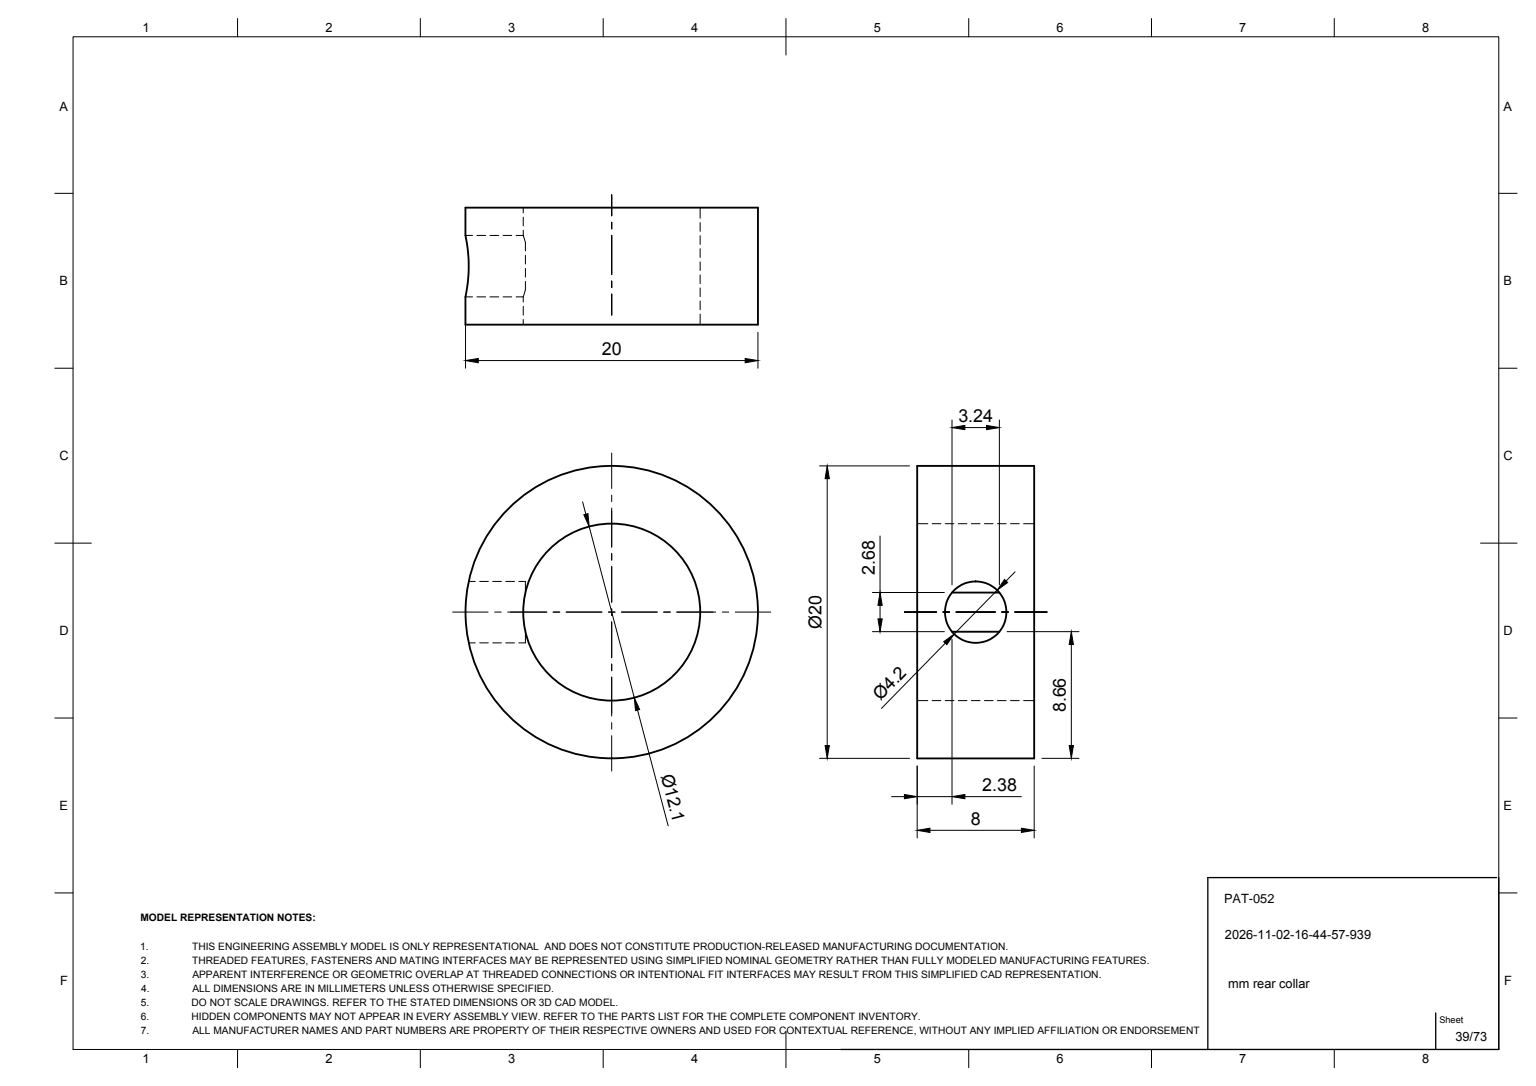
ISO-10303-21;
HEADER;
/* Generated by software containing ST-Developer
 * from STEP Tools, Inc. (www.steptools.com) 
 */

FILE_DESCRIPTION(
/* description */ ('Hand-crank gear train demonstrator'),
/* implementation_level */ '2;1');

FILE_NAME(
/* name */ 'mm rear collar.step',
/* time_stamp */ '2026-10-28T03:22:13-07:00',
/* author */ (''),
/* organization */ (''),
/* preprocessor_version */ 'ST-DEVELOPER v20.2',
/* originating_system */ 'Autodesk Translation Framework v15.17.0.0',
/* authorisation */ '');

FILE_SCHEMA (('AUTOMOTIVE_DESIGN { 1 0 10303 214 3 1 1 }'));
ENDSEC;

DATA;
#10=MECHANICAL_DESIGN_GEOMETRIC_PRESENTATION_REPRESENTATION('',(#1235),#62758);
#891=B_SPLINE_CURVE_WITH_KNOTS('',3,(#26102,#26103,#26104,#26105,#26106,
#26107,#26108,#26109,#26110,#26111),.UNSPECIFIED.,.F.,.F.,(4,2,2,2,4),(0.818088904349178,
0.878131747417164,0.957937926194035,1.03774410497091,1.09778694803889),
 .UNSPECIFIED.);
#892=B_SPLINE_CURVE_WITH_KNOTS('',3,(#26117,#26118,#26119,#26120,#26121,
#26122,#26123,#26124,#26125,#26126,#26127,#26128,#26129,#26130,#26131,#26132,
#26133,#26134),.UNSPECIFIED.,.F.,.F.,(4,2,2,2,2,2,2,2,4),(0.,0.0793616477694785,
0.158723295538957,0.238079516586307,0.317435737633656,0.396791958681006,
0.476148179728355,0.555509827497834,0.634871475267312),.UNSPECIFIED.);
#893=B_SPLINE_CURVE_WITH_KNOTS('',3,(#26135,#26136,#26137,#26138,#26139,
#26140,#26141,#26142,#26143,#26144,#26145,#26146,#26147,#26148,#26149,#26150,
#26151,#26152),.UNSPECIFIED.,.F.,.F.,(4,2,2,2,2,2,2,2,4),(0.634871475267312,
0.714233123036791,0.793594770806269,0.872950991853619,0.952307212900969,
1.03166343394832,1.11101965499567,1.19038130276515,1.26974295053462),
 .UNSPECIFIED.);
#894=B_SPLINE_CURVE_WITH_KNOTS('',3,(#26155,#26156,#26157,#26158,#26159,
#26160,#26161,#26162,#26163,#26164),.UNSPECIFIED.,.F.,.F.,(4,2,2,2,4),(0.179463620219821,
0.239506463287807,0.319312642064678,0.399118820841549,0.459161663909536),
 .UNSPECIFIED.);
#1092=SHAPE_REPRESENTATION_RELATIONSHIP('SRR','None',#63067,#1156);
#1156=ADVANCED_BREP_SHAPE_REPRESENTATION('',(#1311),#62721);
#1235=STYLED_ITEM('',(#63448),#1311);
#1311=MANIFOLD_SOLID_BREP('Body1',#16418);
#1551=FACE_BOUND('',#3723,.T.);
#1552=FACE_BOUND('',#3725,.T.);
#1553=FACE_BOUND('',#3727,.T.);
#1554=FACE_BOUND('',#3729,.T.);
#1902=PLANE('',#18024);
#1903=PLANE('',#18029);
#1904=PLANE('',#18036);
#1905=PLANE('',#18037);
#2574=FACE_OUTER_BOUND('',#3719,.T.);
#2575=FACE_OUTER_BOUND('',#3720,.T.);
#2576=FACE_OUTER_BOUND('',#3721,.T.);
#2577=FACE_OUTER_BOUND('',#3722,.T.);
#2578=FACE_OUTER_BOUND('',#3724,.T.);
#2579=FACE_OUTER_BOUND('',#3726,.T.);
#2580=FACE_OUTER_BOUND('',#3728,.T.);
#3719=EDGE_LOOP('',(#12805,#12806));
#3720=EDGE_LOOP('',(#12807,#12808,#12809,#12810,#12811,#12812,#12813,#12814,
#12815));
#3721=EDGE_LOOP('',(#12816,#12817,#12818));
#3722=EDGE_LOOP('',(#12819,#12820,#12821,#12822));
#3723=EDGE_LOOP('',(#12823,#12824,#12825,#12826));
#3724=EDGE_LOOP('',(#12827,#12828,#12829,#12830));
#3725=EDGE_LOOP('',(#12831,#12832));
#3726=EDGE_LOOP('',(#12833));
#3727=EDGE_LOOP('',(#12834));
#3728=EDGE_LOOP('',(#12835));
#3729=EDGE_LOOP('',(#12836));
#4871=LINE('',#26098,#6003);
#4872=LINE('',#26115,#6004);
#4873=LINE('',#26166,#6005);
#4874=LINE('',#26171,#6006);
#4875=LINE('',#26177,#6007);
#6003=VECTOR('',#21150,1.);
#6004=VECTOR('',#21157,0.21);
#6005=VECTOR('',#21162,1.);
#6006=VECTOR('',#21167,0.605);
#6007=VECTOR('',#21174,1.);
#6918=CIRCLE('',#18025,0.21);
#6919=CIRCLE('',#18027,0.21);
#6920=CIRCLE('',#18028,0.21);
#6921=CIRCLE('',#18031,0.605);
#6922=CIRCLE('',#18032,0.605);
#6923=CIRCLE('',#18034,1.);
#6924=CIRCLE('',#18035,1.);
#7883=VERTEX_POINT('',#26096);
#7884=VERTEX_POINT('',#26097);
#7885=VERTEX_POINT('',#26101);
#7886=VERTEX_POINT('',#26112);
#7887=VERTEX_POINT('',#26114);
#7888=VERTEX_POINT('',#26116);
#7889=VERTEX_POINT('',#26153);
#7890=VERTEX_POINT('',#26168);
#7891=VERTEX_POINT('',#26170);
#7892=VERTEX_POINT('',#26174);
#7893=VERTEX_POINT('',#26176);
#9654=EDGE_CURVE('',#7883,#7884,#4871,.T.);
#9655=EDGE_CURVE('',#7883,#7884,#6918,.T.);
#9656=EDGE_CURVE('',#7885,#7883,#891,.T.);
#9657=EDGE_CURVE('',#7886,#7885,#6919,.T.);
#9658=EDGE_CURVE('',#7886,#7887,#4872,.T.);
#9659=EDGE_CURVE('',#7888,#7887,#892,.T.);
#9660=EDGE_CURVE('',#7887,#7888,#893,.T.);
#9661=EDGE_CURVE('',#7889,#7886,#6920,.T.);
#9662=EDGE_CURVE('',#7884,#7889,#894,.T.);
#9663=EDGE_CURVE('',#7889,#7885,#4873,.T.);
#9664=EDGE_CURVE('',#7890,#7890,#6921,.T.);
#9665=EDGE_CURVE('',#7890,#7891,#4874,.T.);
#9666=EDGE_CURVE('',#7891,#7891,#6922,.T.);
#9667=EDGE_CURVE('',#7892,#7892,#6923,.T.);
#9668=EDGE_CURVE('',#7892,#7893,#4875,.T.);
#9669=EDGE_CURVE('',#7893,#7893,#6924,.T.);
#12805=ORIENTED_EDGE('',*,*,#9654,.F.);
#12806=ORIENTED_EDGE('',*,*,#9655,.T.);
#12807=ORIENTED_EDGE('',*,*,#9656,.F.);
#12808=ORIENTED_EDGE('',*,*,#9657,.F.);
#12809=ORIENTED_EDGE('',*,*,#9658,.T.);
#12810=ORIENTED_EDGE('',*,*,#9659,.F.);
#12811=ORIENTED_EDGE('',*,*,#9660,.F.);
#12812=ORIENTED_EDGE('',*,*,#9658,.F.);
#12813=ORIENTED_EDGE('',*,*,#9661,.F.);
#12814=ORIENTED_EDGE('',*,*,#9662,.F.);
#12815=ORIENTED_EDGE('',*,*,#9655,.F.);
#12816=ORIENTED_EDGE('',*,*,#9663,.F.);
#12817=ORIENTED_EDGE('',*,*,#9661,.T.);
#12818=ORIENTED_EDGE('',*,*,#9657,.T.);
#12819=ORIENTED_EDGE('',*,*,#9664,.F.);
#12820=ORIENTED_EDGE('',*,*,#9665,.T.);
#12821=ORIENTED_EDGE('',*,*,#9666,.T.);
#12822=ORIENTED_EDGE('',*,*,#9665,.F.);
#12823=ORIENTED_EDGE('',*,*,#9662,.T.);
#12824=ORIENTED_EDGE('',*,*,#9663,.T.);
#12825=ORIENTED_EDGE('',*,*,#9656,.T.);
#12826=ORIENTED_EDGE('',*,*,#9654,.T.);
#12827=ORIENTED_EDGE('',*,*,#9667,.F.);
#12828=ORIENTED_EDGE('',*,*,#9668,.T.);
#12829=ORIENTED_EDGE('',*,*,#9669,.T.);
#12830=ORIENTED_EDGE('',*,*,#9668,.F.);
#12831=ORIENTED_EDGE('',*,*,#9659,.T.);
#12832=ORIENTED_EDGE('',*,*,#9660,.T.);
#12833=ORIENTED_EDGE('',*,*,#9667,.T.);
#12834=ORIENTED_EDGE('',*,*,#9664,.T.);
#12835=ORIENTED_EDGE('',*,*,#9669,.F.);
#12836=ORIENTED_EDGE('',*,*,#9666,.F.);
#15298=CYLINDRICAL_SURFACE('',#18026,0.21);
#15299=CYLINDRICAL_SURFACE('',#18030,0.605);
#15300=CYLINDRICAL_SURFACE('',#18033,1.);
#15884=ADVANCED_FACE('',(#2574),#1902,.T.);
#15885=ADVANCED_FACE('',(#2575),#15298,.F.);
#15886=ADVANCED_FACE('',(#2576),#1903,.T.);
#15887=ADVANCED_FACE('',(#2577,#1551),#15299,.F.);
#15888=ADVANCED_FACE('',(#2578,#1552),#15300,.T.);
#15889=ADVANCED_FACE('',(#2579,#1553),#1904,.T.);
#15890=ADVANCED_FACE('',(#2580,#1554),#1905,.F.);
#16418=CLOSED_SHELL('',(#15884,#15885,#15886,#15887,#15888,#15889,#15890));
#18023=AXIS2_PLACEMENT_3D('',#26094,#21146,#21147);
#18024=AXIS2_PLACEMENT_3D('',#26095,#21148,#21149);
#18025=AXIS2_PLACEMENT_3D('',#26099,#21151,#21152);
#18026=AXIS2_PLACEMENT_3D('',#26100,#21153,#21154);
#18027=AXIS2_PLACEMENT_3D('',#26113,#21155,#21156);
#18028=AXIS2_PLACEMENT_3D('',#26154,#21158,#21159);
#18029=AXIS2_PLACEMENT_3D('',#26165,#21160,#21161);
#18030=AXIS2_PLACEMENT_3D('',#26167,#21163,#21164);
#18031=AXIS2_PLACEMENT_3D('',#26169,#21165,#21166);
#18032=AXIS2_PLACEMENT_3D('',#26172,#21168,#21169);
#18033=AXIS2_PLACEMENT_3D('',#26173,#21170,#21171);
#18034=AXIS2_PLACEMENT_3D('',#26175,#21172,#21173);
#18035=AXIS2_PLACEMENT_3D('',#26178,#21175,#21176);
#18036=AXIS2_PLACEMENT_3D('',#26179,#21177,#21178);
#18037=AXIS2_PLACEMENT_3D('',#26180,#21179,#21180);
#21146=DIRECTION('axis',(0.,0.,1.));
#21147=DIRECTION('refdir',(1.,0.,0.));
#21148=DIRECTION('center_axis',(0.,0.,1.));
#21149=DIRECTION('ref_axis',(1.,0.,0.));
#21150=DIRECTION('',(0.,1.,0.));
#21151=DIRECTION('center_axis',(0.,0.,1.));
#21152=DIRECTION('ref_axis',(1.,0.,0.));
#21153=DIRECTION('center_axis',(0.,0.,1.));
#21154=DIRECTION('ref_axis',(1.,0.,0.));
#21155=DIRECTION('center_axis',(0.,0.,1.));
#21156=DIRECTION('ref_axis',(1.,0.,0.));
#21157=DIRECTION('',(0.,0.,1.));
#21158=DIRECTION('center_axis',(0.,0.,1.));
#21159=DIRECTION('ref_axis',(1.,0.,0.));
#21160=DIRECTION('center_axis',(0.,0.,1.));
#21161=DIRECTION('ref_axis',(1.,0.,0.));
#21162=DIRECTION('',(0.,-1.,0.));
#21163=DIRECTION('center_axis',(0.,1.,0.));
#21164=DIRECTION('ref_axis',(1.,0.,0.));
#21165=DIRECTION('center_axis',(0.,-1.,0.));
#21166=DIRECTION('ref_axis',(1.,0.,0.));
#21167=DIRECTION('',(0.,-1.,0.));
#21168=DIRECTION('center_axis',(0.,-1.,0.));
#21169=DIRECTION('ref_axis',(1.,0.,0.));
#21170=DIRECTION('center_axis',(0.,1.,0.));
#21171=DIRECTION('ref_axis',(1.,0.,0.));
#21172=DIRECTION('center_axis',(0.,1.,0.));
#21173=DIRECTION('ref_axis',(1.,0.,0.));
#21174=DIRECTION('',(0.,-1.,0.));
#21175=DIRECTION('center_axis',(0.,1.,0.));
#21176=DIRECTION('ref_axis',(1.,0.,0.));
#21177=DIRECTION('center_axis',(0.,1.,0.));
#21178=DIRECTION('ref_axis',(1.,0.,0.));
#21179=DIRECTION('center_axis',(0.,1.,0.));
#21180=DIRECTION('ref_axis',(1.,0.,0.));
#26094=CARTESIAN_POINT('',(0.,0.,0.));
#26095=CARTESIAN_POINT('Origin',(0.,-3.2,9.59));
#26096=CARTESIAN_POINT('',(0.133884278389952,-3.36178689687364,9.59));
#26097=CARTESIAN_POINT('',(0.133884278389952,-3.03821310312636,9.59));
#26098=CARTESIAN_POINT('',(0.133884278389952,-3.6,9.59));
#26099=CARTESIAN_POINT('Origin',(0.,-3.2,9.59));
#26100=CARTESIAN_POINT('Origin',(0.,-3.2,9.59));
#26101=CARTESIAN_POINT('',(-0.133884278389952,-3.36178689687364,9.59));
#26102=CARTESIAN_POINT('Ctrl Pts',(-0.133884278389951,-3.36178689687364,
9.59));
#26103=CARTESIAN_POINT('Ctrl Pts',(-0.118254395260798,-3.37472116821763,
9.59354677224418));
#26104=CARTESIAN_POINT('Ctrl Pts',(-0.100109787682297,-3.38579931658744,
9.59698224789957));
#26105=CARTESIAN_POINT('Ctrl Pts',(-0.054829872132519,-3.40463856105443,
9.6030741628997));
#26106=CARTESIAN_POINT('Ctrl Pts',(-0.0266020595922904,-3.41,9.605));
#26107=CARTESIAN_POINT('Ctrl Pts',(0.0266020595922903,-3.41,9.605));
#26108=CARTESIAN_POINT('Ctrl Pts',(0.0548298721325192,-3.40463856105443,
9.6030741628997));
#26109=CARTESIAN_POINT('Ctrl Pts',(0.100109787682297,-3.38579931658744,
9.59698224789957));
#26110=CARTESIAN_POINT('Ctrl Pts',(0.118254395260799,-3.37472116821763,
9.59354677224418));
#26111=CARTESIAN_POINT('Ctrl Pts',(0.133884278389952,-3.36178689687364,
9.59));
#26112=CARTESIAN_POINT('',(-0.21,-3.2,9.59));
#26113=CARTESIAN_POINT('Origin',(0.,-3.2,9.59));
#26114=CARTESIAN_POINT('',(-0.21,-3.2,9.97770138590472));
#26115=CARTESIAN_POINT('',(-0.21,-3.2,9.59));
#26116=CARTESIAN_POINT('',(0.21,-3.2,9.97770138590472));
#26117=CARTESIAN_POINT('Ctrl Pts',(0.21,-3.2,9.97770138590472));
#26118=CARTESIAN_POINT('Ctrl Pts',(0.21,-3.22645388258983,9.97770138590472));
#26119=CARTESIAN_POINT('Ctrl Pts',(0.204697017125528,-3.25461525830869,
9.97888646613217));
#26120=CARTESIAN_POINT('Ctrl Pts',(0.183241751515529,-3.30633042130174,
9.98312869991147));
#26121=CARTESIAN_POINT('Ctrl Pts',(0.167093586802906,-3.32989126129544,
9.98612044796649));
#26122=CARTESIAN_POINT('Ctrl Pts',(0.129892533236543,-3.36709231486181,
9.99170645156379));
#26123=CARTESIAN_POINT('Ctrl Pts',(0.106331154992714,-3.38324147510569,
9.99466914446598));
#26124=CARTESIAN_POINT('Ctrl Pts',(0.0546141143983532,-3.40469746372443,
9.99884449237241));
#26125=CARTESIAN_POINT('Ctrl Pts',(0.0264520736824499,-3.41,10.));
#26126=CARTESIAN_POINT('Ctrl Pts',(-0.0264520736824498,-3.41,10.));
#26127=CARTESIAN_POINT('Ctrl Pts',(-0.0546141143983531,-3.40469746372443,
9.99884449237241));
#26128=CARTESIAN_POINT('Ctrl Pts',(-0.106331154992714,-3.38324147510569,
9.99466914446598));
#26129=CARTESIAN_POINT('Ctrl Pts',(-0.129892533236543,-3.36709231486181,
9.99170645156379));
#26130=CARTESIAN_POINT('Ctrl Pts',(-0.167093586802906,-3.32989126129544,
9.98612044796649));
#26131=CARTESIAN_POINT('Ctrl Pts',(-0.183241751515529,-3.30633042130174,
9.98312869991147));
#26132=CARTESIAN_POINT('Ctrl Pts',(-0.204697017125528,-3.25461525830869,
9.97888646613217));
#26133=CARTESIAN_POINT('Ctrl Pts',(-0.21,-3.22645388258983,9.97770138590472));
#26134=CARTESIAN_POINT('Ctrl Pts',(-0.21,-3.2,9.97770138590472));
#26135=CARTESIAN_POINT('Ctrl Pts',(-0.21,-3.2,9.97770138590472));
#26136=CARTESIAN_POINT('Ctrl Pts',(-0.21,-3.17354611741017,9.97770138590472));
#26137=CARTESIAN_POINT('Ctrl Pts',(-0.204697017125528,-3.14538474169131,
9.97888646613217));
#26138=CARTESIAN_POINT('Ctrl Pts',(-0.183241751515529,-3.09366957869826,
9.98312869991147));
#26139=CARTESIAN_POINT('Ctrl Pts',(-0.167093586802906,-3.07010873870456,
9.98612044796649));
#26140=CARTESIAN_POINT('Ctrl Pts',(-0.129892533236543,-3.03290768513819,
9.99170645156379));
#26141=CARTESIAN_POINT('Ctrl Pts',(-0.106331154992714,-3.01675852489431,
9.99466914446598));
#26142=CARTESIAN_POINT('Ctrl Pts',(-0.0546141143983532,-2.99530253627557,
9.99884449237241));
#26143=CARTESIAN_POINT('Ctrl Pts',(-0.0264520736824499,-2.99,10.));
#26144=CARTESIAN_POINT('Ctrl Pts',(0.0264520736824498,-2.99,10.));
#26145=CARTESIAN_POINT('Ctrl Pts',(0.0546141143983531,-2.99530253627557,
9.99884449237241));
#26146=CARTESIAN_POINT('Ctrl Pts',(0.106331154992714,-3.01675852489431,
9.99466914446598));
#26147=CARTESIAN_POINT('Ctrl Pts',(0.129892533236543,-3.03290768513819,
9.99170645156379));
#26148=CARTESIAN_POINT('Ctrl Pts',(0.167093586802906,-3.07010873870456,
9.98612044796649));
#26149=CARTESIAN_POINT('Ctrl Pts',(0.183241751515529,-3.09366957869826,
9.98312869991147));
#26150=CARTESIAN_POINT('Ctrl Pts',(0.204697017125528,-3.14538474169131,
9.97888646613217));
#26151=CARTESIAN_POINT('Ctrl Pts',(0.21,-3.17354611741017,9.97770138590472));
#26152=CARTESIAN_POINT('Ctrl Pts',(0.21,-3.2,9.97770138590472));
#26153=CARTESIAN_POINT('',(-0.133884278389952,-3.03821310312636,9.59));
#26154=CARTESIAN_POINT('Origin',(0.,-3.2,9.59));
#26155=CARTESIAN_POINT('Ctrl Pts',(0.133884278389952,-3.03821310312636,
9.59));
#26156=CARTESIAN_POINT('Ctrl Pts',(0.118254395260799,-3.02527883178237,
9.59354677224418));
#26157=CARTESIAN_POINT('Ctrl Pts',(0.100109787682297,-3.01420068341256,
9.59698224789957));
#26158=CARTESIAN_POINT('Ctrl Pts',(0.054829872132519,-2.99536143894557,
9.6030741628997));
#26159=CARTESIAN_POINT('Ctrl Pts',(0.0266020595922904,-2.99,9.605));
#26160=CARTESIAN_POINT('Ctrl Pts',(-0.0266020595922903,-2.99,9.605));
#26161=CARTESIAN_POINT('Ctrl Pts',(-0.054829872132519,-2.99536143894557,
9.6030741628997));
#26162=CARTESIAN_POINT('Ctrl Pts',(-0.100109787682297,-3.01420068341256,
9.59698224789957));
#26163=CARTESIAN_POINT('Ctrl Pts',(-0.118254395260798,-3.02527883178237,
9.59354677224418));
#26164=CARTESIAN_POINT('Ctrl Pts',(-0.133884278389952,-3.03821310312636,
9.59));
#26165=CARTESIAN_POINT('Origin',(0.,-3.2,9.59));
#26166=CARTESIAN_POINT('',(-0.133884278389952,-3.6,9.59));
#26167=CARTESIAN_POINT('Origin',(0.,-3.6,9.));
#26168=CARTESIAN_POINT('',(-0.605,-2.8,9.));
#26169=CARTESIAN_POINT('Origin',(0.,-2.8,9.));
#26170=CARTESIAN_POINT('',(-0.605,-3.6,9.));
#26171=CARTESIAN_POINT('',(-0.605,-3.6,9.));
#26172=CARTESIAN_POINT('Origin',(0.,-3.6,9.));
#26173=CARTESIAN_POINT('Origin',(0.,-3.6,9.));
#26174=CARTESIAN_POINT('',(-1.,-2.8,9.));
#26175=CARTESIAN_POINT('Origin',(0.,-2.8,9.));
#26176=CARTESIAN_POINT('',(-1.,-3.6,9.));
#26177=CARTESIAN_POINT('',(-1.,-3.6,9.));
#26178=CARTESIAN_POINT('Origin',(0.,-3.6,9.));
#26179=CARTESIAN_POINT('Origin',(0.,-2.8,9.));
#26180=CARTESIAN_POINT('Origin',(0.,-3.6,9.));
#62647=UNCERTAINTY_MEASURE_WITH_UNIT(LENGTH_MEASURE(0.001),#62759,
'DISTANCE_ACCURACY_VALUE',
'Maximum model space distance between geometric entities at asserted c
onnectivities');
#62684=UNCERTAINTY_MEASURE_WITH_UNIT(LENGTH_MEASURE(0.001),#62759,
'DISTANCE_ACCURACY_VALUE',
'Maximum model space distance between geometric entities at asserted c
onnectivities');
#62721=(
GEOMETRIC_REPRESENTATION_CONTEXT(3)
GLOBAL_UNCERTAINTY_ASSIGNED_CONTEXT((#62647))
GLOBAL_UNIT_ASSIGNED_CONTEXT((#62759,#62761,#62762))
REPRESENTATION_CONTEXT('','3D')
);
#62758=(
GEOMETRIC_REPRESENTATION_CONTEXT(3)
GLOBAL_UNCERTAINTY_ASSIGNED_CONTEXT((#62684))
GLOBAL_UNIT_ASSIGNED_CONTEXT((#62759,#62761,#62762))
REPRESENTATION_CONTEXT('','3D')
);
#62759=(
LENGTH_UNIT()
NAMED_UNIT(*)
SI_UNIT(.CENTI.,.METRE.)
);
#62761=(
NAMED_UNIT(*)
PLANE_ANGLE_UNIT()
SI_UNIT($,.RADIAN.)
);
#62762=(
NAMED_UNIT(*)
SI_UNIT($,.STERADIAN.)
SOLID_ANGLE_UNIT()
);
#62799=SHAPE_DEFINITION_REPRESENTATION(#62882,#63067);
#62882=PRODUCT_DEFINITION_SHAPE('',$,#63141);
#63067=SHAPE_REPRESENTATION('',(#18023),#62721);
#63104=PRODUCT_DEFINITION_CONTEXT('part definition',#63325,'design');
#63141=PRODUCT_DEFINITION('mm rear collar','mm rear collar',#63214,#63104);
#63214=PRODUCT_DEFINITION_FORMATION('',$,#63363);
#63325=APPLICATION_CONTEXT(
'Core Data for Automotive Mechanical Design Process');
#63326=PRODUCT_CONTEXT('part definition',#63325,'mechanical');
#63363=PRODUCT('mm rear collar','mm rear collar','mm rear collar',(#63326));
#63442=COLOUR_RGB('Light Blue',0.38,0.62,0.78);
#63443=FILL_AREA_STYLE_COLOUR('',#63442);
#63444=FILL_AREA_STYLE('',(#63443));
#63445=SURFACE_STYLE_FILL_AREA(#63444);
#63446=SURFACE_SIDE_STYLE('',(#63445));
#63447=SURFACE_STYLE_USAGE(.BOTH.,#63446);
#63448=PRESENTATION_STYLE_ASSIGNMENT((#63447));
ENDSEC;
END-ISO-10303-21;
